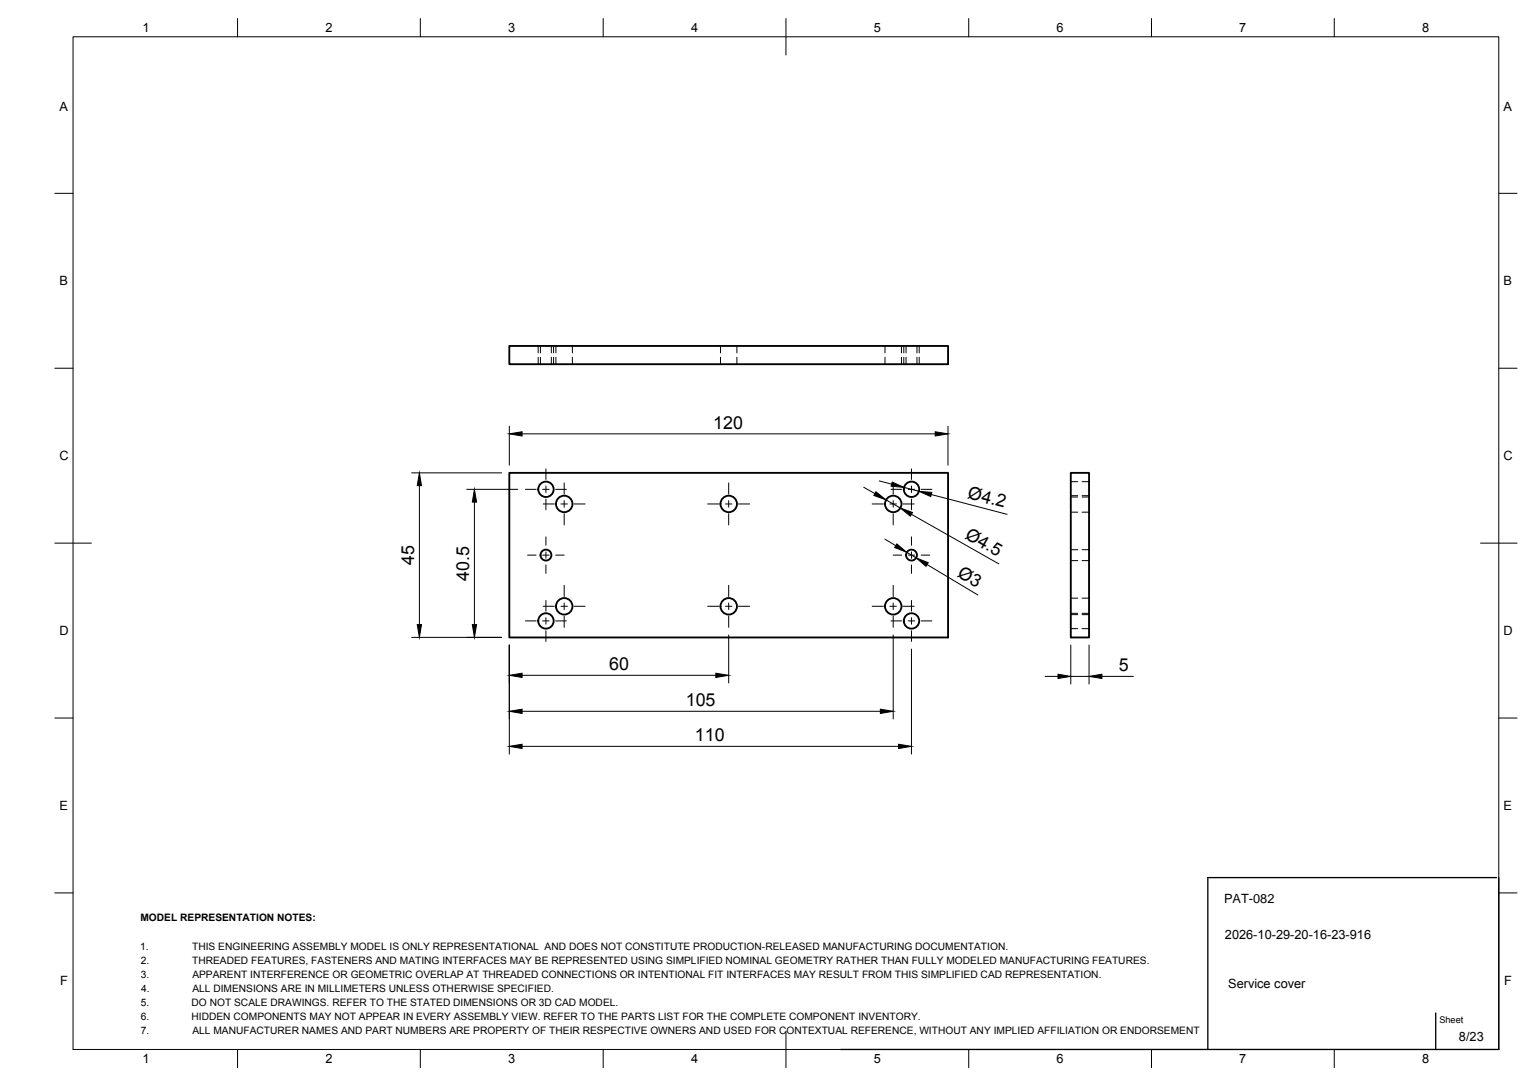
ISO-10303-21;
HEADER;
/* Generated by software containing ST-Developer
 * from STEP Tools, Inc. (www.steptools.com) 
 */

FILE_DESCRIPTION(
/* description */ ('PAT-082'),
/* implementation_level */ '2;1');

FILE_NAME(
/* name */ 'Service cover.step',
/* time_stamp */ '2026-10-29T20:16:13-07:00',
/* author */ (''),
/* organization */ (''),
/* preprocessor_version */ 'ST-DEVELOPER v20.2',
/* originating_system */ 'Autodesk Translation Framework v15.17.0.0',
/* authorisation */ '');

FILE_SCHEMA (('AUTOMOTIVE_DESIGN { 1 0 10303 214 3 1 1 }'));
ENDSEC;

DATA;
#10=MECHANICAL_DESIGN_GEOMETRIC_PRESENTATION_REPRESENTATION('',(#246),#8266);
#202=SHAPE_REPRESENTATION_RELATIONSHIP('SRR','None',#8364,#224);
#224=ADVANCED_BREP_SHAPE_REPRESENTATION('',(#268),#8248);
#246=STYLED_ITEM('',(#8551),#268);
#268=MANIFOLD_SOLID_BREP('Body1',#4586);
#310=FACE_BOUND('',#945,.T.);
#311=FACE_BOUND('',#946,.T.);
#312=FACE_BOUND('',#947,.T.);
#313=FACE_BOUND('',#948,.T.);
#314=FACE_BOUND('',#949,.T.);
#315=FACE_BOUND('',#950,.T.);
#316=FACE_BOUND('',#951,.T.);
#317=FACE_BOUND('',#952,.T.);
#318=FACE_BOUND('',#953,.T.);
#319=FACE_BOUND('',#954,.T.);
#320=FACE_BOUND('',#955,.T.);
#321=FACE_BOUND('',#956,.T.);
#322=FACE_BOUND('',#958,.T.);
#323=FACE_BOUND('',#959,.T.);
#324=FACE_BOUND('',#960,.T.);
#325=FACE_BOUND('',#961,.T.);
#326=FACE_BOUND('',#962,.T.);
#327=FACE_BOUND('',#963,.T.);
#328=FACE_BOUND('',#964,.T.);
#329=FACE_BOUND('',#965,.T.);
#330=FACE_BOUND('',#966,.T.);
#331=FACE_BOUND('',#967,.T.);
#332=FACE_BOUND('',#968,.T.);
#333=FACE_BOUND('',#969,.T.);
#443=PLANE('',#4998);
#444=PLANE('',#4999);
#445=PLANE('',#5000);
#446=PLANE('',#5001);
#447=PLANE('',#5002);
#448=PLANE('',#5003);
#630=FACE_OUTER_BOUND('',#928,.T.);
#631=FACE_OUTER_BOUND('',#929,.T.);
#632=FACE_OUTER_BOUND('',#930,.T.);
#633=FACE_OUTER_BOUND('',#931,.T.);
#634=FACE_OUTER_BOUND('',#932,.T.);
#635=FACE_OUTER_BOUND('',#933,.T.);
#636=FACE_OUTER_BOUND('',#934,.T.);
#637=FACE_OUTER_BOUND('',#935,.T.);
#638=FACE_OUTER_BOUND('',#936,.T.);
#639=FACE_OUTER_BOUND('',#937,.T.);
#640=FACE_OUTER_BOUND('',#938,.T.);
#641=FACE_OUTER_BOUND('',#939,.T.);
#642=FACE_OUTER_BOUND('',#940,.T.);
#643=FACE_OUTER_BOUND('',#941,.T.);
#644=FACE_OUTER_BOUND('',#942,.T.);
#645=FACE_OUTER_BOUND('',#943,.T.);
#646=FACE_OUTER_BOUND('',#944,.T.);
#647=FACE_OUTER_BOUND('',#957,.T.);
#928=EDGE_LOOP('',(#3350,#3351,#3352,#3353));
#929=EDGE_LOOP('',(#3354,#3355,#3356,#3357));
#930=EDGE_LOOP('',(#3358,#3359,#3360,#3361));
#931=EDGE_LOOP('',(#3362,#3363,#3364,#3365));
#932=EDGE_LOOP('',(#3366,#3367,#3368,#3369));
#933=EDGE_LOOP('',(#3370,#3371,#3372,#3373));
#934=EDGE_LOOP('',(#3374,#3375,#3376,#3377));
#935=EDGE_LOOP('',(#3378,#3379,#3380,#3381));
#936=EDGE_LOOP('',(#3382,#3383,#3384,#3385));
#937=EDGE_LOOP('',(#3386,#3387,#3388,#3389));
#938=EDGE_LOOP('',(#3390,#3391,#3392,#3393));
#939=EDGE_LOOP('',(#3394,#3395,#3396,#3397));
#940=EDGE_LOOP('',(#3398,#3399,#3400,#3401));
#941=EDGE_LOOP('',(#3402,#3403,#3404,#3405));
#942=EDGE_LOOP('',(#3406,#3407,#3408,#3409));
#943=EDGE_LOOP('',(#3410,#3411,#3412,#3413));
#944=EDGE_LOOP('',(#3414,#3415,#3416,#3417));
#945=EDGE_LOOP('',(#3418));
#946=EDGE_LOOP('',(#3419));
#947=EDGE_LOOP('',(#3420));
#948=EDGE_LOOP('',(#3421));
#949=EDGE_LOOP('',(#3422));
#950=EDGE_LOOP('',(#3423));
#951=EDGE_LOOP('',(#3424));
#952=EDGE_LOOP('',(#3425));
#953=EDGE_LOOP('',(#3426));
#954=EDGE_LOOP('',(#3427));
#955=EDGE_LOOP('',(#3428));
#956=EDGE_LOOP('',(#3429));
#957=EDGE_LOOP('',(#3430,#3431,#3432,#3433));
#958=EDGE_LOOP('',(#3434));
#959=EDGE_LOOP('',(#3435));
#960=EDGE_LOOP('',(#3436));
#961=EDGE_LOOP('',(#3437));
#962=EDGE_LOOP('',(#3438));
#963=EDGE_LOOP('',(#3439));
#964=EDGE_LOOP('',(#3440));
#965=EDGE_LOOP('',(#3441));
#966=EDGE_LOOP('',(#3442));
#967=EDGE_LOOP('',(#3443));
#968=EDGE_LOOP('',(#3444));
#969=EDGE_LOOP('',(#3445));
#1319=LINE('',#7092,#1674);
#1320=LINE('',#7098,#1675);
#1321=LINE('',#7104,#1676);
#1322=LINE('',#7110,#1677);
#1323=LINE('',#7116,#1678);
#1324=LINE('',#7122,#1679);
#1325=LINE('',#7128,#1680);
#1326=LINE('',#7134,#1681);
#1327=LINE('',#7140,#1682);
#1328=LINE('',#7146,#1683);
#1329=LINE('',#7152,#1684);
#1330=LINE('',#7158,#1685);
#1331=LINE('',#7163,#1686);
#1332=LINE('',#7165,#1687);
#1333=LINE('',#7167,#1688);
#1334=LINE('',#7168,#1689);
#1335=LINE('',#7171,#1690);
#1336=LINE('',#7173,#1691);
#1337=LINE('',#7174,#1692);
#1338=LINE('',#7177,#1693);
#1339=LINE('',#7179,#1694);
#1340=LINE('',#7180,#1695);
#1341=LINE('',#7182,#1696);
#1342=LINE('',#7183,#1697);
#1674=VECTOR('',#5696,0.15);
#1675=VECTOR('',#5703,0.15);
#1676=VECTOR('',#5710,0.225);
#1677=VECTOR('',#5717,0.225);
#1678=VECTOR('',#5724,0.225);
#1679=VECTOR('',#5731,0.225);
#1680=VECTOR('',#5738,0.225);
#1681=VECTOR('',#5745,0.225);
#1682=VECTOR('',#5752,0.21);
#1683=VECTOR('',#5759,0.21);
#1684=VECTOR('',#5766,0.21);
#1685=VECTOR('',#5773,0.21);
#1686=VECTOR('',#5778,1.);
#1687=VECTOR('',#5779,1.);
#1688=VECTOR('',#5780,1.);
#1689=VECTOR('',#5781,1.);
#1690=VECTOR('',#5784,1.);
#1691=VECTOR('',#5785,1.);
#1692=VECTOR('',#5786,1.);
#1693=VECTOR('',#5789,1.);
#1694=VECTOR('',#5790,1.);
#1695=VECTOR('',#5791,1.);
#1696=VECTOR('',#5794,1.);
#1697=VECTOR('',#5795,1.);
#1993=CIRCLE('',#4963,0.15);
#1994=CIRCLE('',#4964,0.15);
#1995=CIRCLE('',#4966,0.15);
#1996=CIRCLE('',#4967,0.15);
#1997=CIRCLE('',#4969,0.225);
#1998=CIRCLE('',#4970,0.225);
#1999=CIRCLE('',#4972,0.225);
#2000=CIRCLE('',#4973,0.225);
#2001=CIRCLE('',#4975,0.225);
#2002=CIRCLE('',#4976,0.225);
#2003=CIRCLE('',#4978,0.225);
#2004=CIRCLE('',#4979,0.225);
#2005=CIRCLE('',#4981,0.225);
#2006=CIRCLE('',#4982,0.225);
#2007=CIRCLE('',#4984,0.225);
#2008=CIRCLE('',#4985,0.225);
#2009=CIRCLE('',#4987,0.21);
#2010=CIRCLE('',#4988,0.21);
#2011=CIRCLE('',#4990,0.21);
#2012=CIRCLE('',#4991,0.21);
#2013=CIRCLE('',#4993,0.21);
#2014=CIRCLE('',#4994,0.21);
#2015=CIRCLE('',#4996,0.21);
#2016=CIRCLE('',#4997,0.21);
#2233=VERTEX_POINT('',#7089);
#2234=VERTEX_POINT('',#7091);
#2235=VERTEX_POINT('',#7095);
#2236=VERTEX_POINT('',#7097);
#2237=VERTEX_POINT('',#7101);
#2238=VERTEX_POINT('',#7103);
#2239=VERTEX_POINT('',#7107);
#2240=VERTEX_POINT('',#7109);
#2241=VERTEX_POINT('',#7113);
#2242=VERTEX_POINT('',#7115);
#2243=VERTEX_POINT('',#7119);
#2244=VERTEX_POINT('',#7121);
#2245=VERTEX_POINT('',#7125);
#2246=VERTEX_POINT('',#7127);
#2247=VERTEX_POINT('',#7131);
#2248=VERTEX_POINT('',#7133);
#2249=VERTEX_POINT('',#7137);
#2250=VERTEX_POINT('',#7139);
#2251=VERTEX_POINT('',#7143);
#2252=VERTEX_POINT('',#7145);
#2253=VERTEX_POINT('',#7149);
#2254=VERTEX_POINT('',#7151);
#2255=VERTEX_POINT('',#7155);
#2256=VERTEX_POINT('',#7157);
#2257=VERTEX_POINT('',#7161);
#2258=VERTEX_POINT('',#7162);
#2259=VERTEX_POINT('',#7164);
#2260=VERTEX_POINT('',#7166);
#2261=VERTEX_POINT('',#7170);
#2262=VERTEX_POINT('',#7172);
#2263=VERTEX_POINT('',#7176);
#2264=VERTEX_POINT('',#7178);
#2651=EDGE_CURVE('',#2233,#2233,#1993,.T.);
#2652=EDGE_CURVE('',#2233,#2234,#1319,.T.);
#2653=EDGE_CURVE('',#2234,#2234,#1994,.T.);
#2654=EDGE_CURVE('',#2235,#2235,#1995,.T.);
#2655=EDGE_CURVE('',#2235,#2236,#1320,.T.);
#2656=EDGE_CURVE('',#2236,#2236,#1996,.T.);
#2657=EDGE_CURVE('',#2237,#2237,#1997,.T.);
#2658=EDGE_CURVE('',#2237,#2238,#1321,.T.);
#2659=EDGE_CURVE('',#2238,#2238,#1998,.T.);
#2660=EDGE_CURVE('',#2239,#2239,#1999,.T.);
#2661=EDGE_CURVE('',#2239,#2240,#1322,.T.);
#2662=EDGE_CURVE('',#2240,#2240,#2000,.T.);
#2663=EDGE_CURVE('',#2241,#2241,#2001,.T.);
#2664=EDGE_CURVE('',#2241,#2242,#1323,.T.);
#2665=EDGE_CURVE('',#2242,#2242,#2002,.T.);
#2666=EDGE_CURVE('',#2243,#2243,#2003,.T.);
#2667=EDGE_CURVE('',#2243,#2244,#1324,.T.);
#2668=EDGE_CURVE('',#2244,#2244,#2004,.T.);
#2669=EDGE_CURVE('',#2245,#2245,#2005,.T.);
#2670=EDGE_CURVE('',#2245,#2246,#1325,.T.);
#2671=EDGE_CURVE('',#2246,#2246,#2006,.T.);
#2672=EDGE_CURVE('',#2247,#2247,#2007,.T.);
#2673=EDGE_CURVE('',#2247,#2248,#1326,.T.);
#2674=EDGE_CURVE('',#2248,#2248,#2008,.T.);
#2675=EDGE_CURVE('',#2249,#2249,#2009,.T.);
#2676=EDGE_CURVE('',#2249,#2250,#1327,.T.);
#2677=EDGE_CURVE('',#2250,#2250,#2010,.T.);
#2678=EDGE_CURVE('',#2251,#2251,#2011,.T.);
#2679=EDGE_CURVE('',#2251,#2252,#1328,.T.);
#2680=EDGE_CURVE('',#2252,#2252,#2012,.T.);
#2681=EDGE_CURVE('',#2253,#2253,#2013,.T.);
#2682=EDGE_CURVE('',#2253,#2254,#1329,.T.);
#2683=EDGE_CURVE('',#2254,#2254,#2014,.T.);
#2684=EDGE_CURVE('',#2255,#2255,#2015,.T.);
#2685=EDGE_CURVE('',#2255,#2256,#1330,.T.);
#2686=EDGE_CURVE('',#2256,#2256,#2016,.T.);
#2687=EDGE_CURVE('',#2257,#2258,#1331,.T.);
#2688=EDGE_CURVE('',#2258,#2259,#1332,.T.);
#2689=EDGE_CURVE('',#2260,#2259,#1333,.T.);
#2690=EDGE_CURVE('',#2257,#2260,#1334,.T.);
#2691=EDGE_CURVE('',#2261,#2257,#1335,.T.);
#2692=EDGE_CURVE('',#2262,#2260,#1336,.T.);
#2693=EDGE_CURVE('',#2261,#2262,#1337,.T.);
#2694=EDGE_CURVE('',#2263,#2261,#1338,.T.);
#2695=EDGE_CURVE('',#2264,#2262,#1339,.T.);
#2696=EDGE_CURVE('',#2263,#2264,#1340,.T.);
#2697=EDGE_CURVE('',#2258,#2263,#1341,.T.);
#2698=EDGE_CURVE('',#2259,#2264,#1342,.T.);
#3350=ORIENTED_EDGE('',*,*,#2651,.F.);
#3351=ORIENTED_EDGE('',*,*,#2652,.T.);
#3352=ORIENTED_EDGE('',*,*,#2653,.F.);
#3353=ORIENTED_EDGE('',*,*,#2652,.F.);
#3354=ORIENTED_EDGE('',*,*,#2654,.F.);
#3355=ORIENTED_EDGE('',*,*,#2655,.T.);
#3356=ORIENTED_EDGE('',*,*,#2656,.F.);
#3357=ORIENTED_EDGE('',*,*,#2655,.F.);
#3358=ORIENTED_EDGE('',*,*,#2657,.F.);
#3359=ORIENTED_EDGE('',*,*,#2658,.T.);
#3360=ORIENTED_EDGE('',*,*,#2659,.F.);
#3361=ORIENTED_EDGE('',*,*,#2658,.F.);
#3362=ORIENTED_EDGE('',*,*,#2660,.F.);
#3363=ORIENTED_EDGE('',*,*,#2661,.T.);
#3364=ORIENTED_EDGE('',*,*,#2662,.F.);
#3365=ORIENTED_EDGE('',*,*,#2661,.F.);
#3366=ORIENTED_EDGE('',*,*,#2663,.F.);
#3367=ORIENTED_EDGE('',*,*,#2664,.T.);
#3368=ORIENTED_EDGE('',*,*,#2665,.F.);
#3369=ORIENTED_EDGE('',*,*,#2664,.F.);
#3370=ORIENTED_EDGE('',*,*,#2666,.F.);
#3371=ORIENTED_EDGE('',*,*,#2667,.T.);
#3372=ORIENTED_EDGE('',*,*,#2668,.F.);
#3373=ORIENTED_EDGE('',*,*,#2667,.F.);
#3374=ORIENTED_EDGE('',*,*,#2669,.F.);
#3375=ORIENTED_EDGE('',*,*,#2670,.T.);
#3376=ORIENTED_EDGE('',*,*,#2671,.F.);
#3377=ORIENTED_EDGE('',*,*,#2670,.F.);
#3378=ORIENTED_EDGE('',*,*,#2672,.F.);
#3379=ORIENTED_EDGE('',*,*,#2673,.T.);
#3380=ORIENTED_EDGE('',*,*,#2674,.F.);
#3381=ORIENTED_EDGE('',*,*,#2673,.F.);
#3382=ORIENTED_EDGE('',*,*,#2675,.F.);
#3383=ORIENTED_EDGE('',*,*,#2676,.T.);
#3384=ORIENTED_EDGE('',*,*,#2677,.F.);
#3385=ORIENTED_EDGE('',*,*,#2676,.F.);
#3386=ORIENTED_EDGE('',*,*,#2678,.F.);
#3387=ORIENTED_EDGE('',*,*,#2679,.T.);
#3388=ORIENTED_EDGE('',*,*,#2680,.F.);
#3389=ORIENTED_EDGE('',*,*,#2679,.F.);
#3390=ORIENTED_EDGE('',*,*,#2681,.F.);
#3391=ORIENTED_EDGE('',*,*,#2682,.T.);
#3392=ORIENTED_EDGE('',*,*,#2683,.F.);
#3393=ORIENTED_EDGE('',*,*,#2682,.F.);
#3394=ORIENTED_EDGE('',*,*,#2684,.F.);
#3395=ORIENTED_EDGE('',*,*,#2685,.T.);
#3396=ORIENTED_EDGE('',*,*,#2686,.F.);
#3397=ORIENTED_EDGE('',*,*,#2685,.F.);
#3398=ORIENTED_EDGE('',*,*,#2687,.T.);
#3399=ORIENTED_EDGE('',*,*,#2688,.T.);
#3400=ORIENTED_EDGE('',*,*,#2689,.F.);
#3401=ORIENTED_EDGE('',*,*,#2690,.F.);
#3402=ORIENTED_EDGE('',*,*,#2691,.T.);
#3403=ORIENTED_EDGE('',*,*,#2690,.T.);
#3404=ORIENTED_EDGE('',*,*,#2692,.F.);
#3405=ORIENTED_EDGE('',*,*,#2693,.F.);
#3406=ORIENTED_EDGE('',*,*,#2694,.T.);
#3407=ORIENTED_EDGE('',*,*,#2693,.T.);
#3408=ORIENTED_EDGE('',*,*,#2695,.F.);
#3409=ORIENTED_EDGE('',*,*,#2696,.F.);
#3410=ORIENTED_EDGE('',*,*,#2697,.T.);
#3411=ORIENTED_EDGE('',*,*,#2696,.T.);
#3412=ORIENTED_EDGE('',*,*,#2698,.F.);
#3413=ORIENTED_EDGE('',*,*,#2688,.F.);
#3414=ORIENTED_EDGE('',*,*,#2698,.T.);
#3415=ORIENTED_EDGE('',*,*,#2695,.T.);
#3416=ORIENTED_EDGE('',*,*,#2692,.T.);
#3417=ORIENTED_EDGE('',*,*,#2689,.T.);
#3418=ORIENTED_EDGE('',*,*,#2656,.T.);
#3419=ORIENTED_EDGE('',*,*,#2686,.T.);
#3420=ORIENTED_EDGE('',*,*,#2683,.T.);
#3421=ORIENTED_EDGE('',*,*,#2680,.T.);
#3422=ORIENTED_EDGE('',*,*,#2677,.T.);
#3423=ORIENTED_EDGE('',*,*,#2674,.T.);
#3424=ORIENTED_EDGE('',*,*,#2671,.T.);
#3425=ORIENTED_EDGE('',*,*,#2668,.T.);
#3426=ORIENTED_EDGE('',*,*,#2665,.T.);
#3427=ORIENTED_EDGE('',*,*,#2662,.T.);
#3428=ORIENTED_EDGE('',*,*,#2659,.T.);
#3429=ORIENTED_EDGE('',*,*,#2653,.T.);
#3430=ORIENTED_EDGE('',*,*,#2697,.F.);
#3431=ORIENTED_EDGE('',*,*,#2687,.F.);
#3432=ORIENTED_EDGE('',*,*,#2691,.F.);
#3433=ORIENTED_EDGE('',*,*,#2694,.F.);
#3434=ORIENTED_EDGE('',*,*,#2654,.T.);
#3435=ORIENTED_EDGE('',*,*,#2684,.T.);
#3436=ORIENTED_EDGE('',*,*,#2681,.T.);
#3437=ORIENTED_EDGE('',*,*,#2678,.T.);
#3438=ORIENTED_EDGE('',*,*,#2675,.T.);
#3439=ORIENTED_EDGE('',*,*,#2672,.T.);
#3440=ORIENTED_EDGE('',*,*,#2669,.T.);
#3441=ORIENTED_EDGE('',*,*,#2666,.T.);
#3442=ORIENTED_EDGE('',*,*,#2663,.T.);
#3443=ORIENTED_EDGE('',*,*,#2660,.T.);
#3444=ORIENTED_EDGE('',*,*,#2657,.T.);
#3445=ORIENTED_EDGE('',*,*,#2651,.T.);
#4240=CYLINDRICAL_SURFACE('',#4962,0.15);
#4241=CYLINDRICAL_SURFACE('',#4965,0.15);
#4242=CYLINDRICAL_SURFACE('',#4968,0.225);
#4243=CYLINDRICAL_SURFACE('',#4971,0.225);
#4244=CYLINDRICAL_SURFACE('',#4974,0.225);
#4245=CYLINDRICAL_SURFACE('',#4977,0.225);
#4246=CYLINDRICAL_SURFACE('',#4980,0.225);
#4247=CYLINDRICAL_SURFACE('',#4983,0.225);
#4248=CYLINDRICAL_SURFACE('',#4986,0.21);
#4249=CYLINDRICAL_SURFACE('',#4989,0.21);
#4250=CYLINDRICAL_SURFACE('',#4992,0.21);
#4251=CYLINDRICAL_SURFACE('',#4995,0.21);
#4369=ADVANCED_FACE('',(#630),#4240,.F.);
#4370=ADVANCED_FACE('',(#631),#4241,.F.);
#4371=ADVANCED_FACE('',(#632),#4242,.F.);
#4372=ADVANCED_FACE('',(#633),#4243,.F.);
#4373=ADVANCED_FACE('',(#634),#4244,.F.);
#4374=ADVANCED_FACE('',(#635),#4245,.F.);
#4375=ADVANCED_FACE('',(#636),#4246,.F.);
#4376=ADVANCED_FACE('',(#637),#4247,.F.);
#4377=ADVANCED_FACE('',(#638),#4248,.F.);
#4378=ADVANCED_FACE('',(#639),#4249,.F.);
#4379=ADVANCED_FACE('',(#640),#4250,.F.);
#4380=ADVANCED_FACE('',(#641),#4251,.F.);
#4381=ADVANCED_FACE('',(#642),#443,.T.);
#4382=ADVANCED_FACE('',(#643),#444,.T.);
#4383=ADVANCED_FACE('',(#644),#445,.T.);
#4384=ADVANCED_FACE('',(#645),#446,.T.);
#4385=ADVANCED_FACE('',(#646,#310,#311,#312,#313,#314,#315,#316,#317,#318,
#319,#320,#321),#447,.T.);
#4386=ADVANCED_FACE('',(#647,#322,#323,#324,#325,#326,#327,#328,#329,#330,
#331,#332,#333),#448,.F.);
#4586=CLOSED_SHELL('',(#4369,#4370,#4371,#4372,#4373,#4374,#4375,#4376,
#4377,#4378,#4379,#4380,#4381,#4382,#4383,#4384,#4385,#4386));
#4961=AXIS2_PLACEMENT_3D('',#7087,#5690,#5691);
#4962=AXIS2_PLACEMENT_3D('',#7088,#5692,#5693);
#4963=AXIS2_PLACEMENT_3D('',#7090,#5694,#5695);
#4964=AXIS2_PLACEMENT_3D('',#7093,#5697,#5698);
#4965=AXIS2_PLACEMENT_3D('',#7094,#5699,#5700);
#4966=AXIS2_PLACEMENT_3D('',#7096,#5701,#5702);
#4967=AXIS2_PLACEMENT_3D('',#7099,#5704,#5705);
#4968=AXIS2_PLACEMENT_3D('',#7100,#5706,#5707);
#4969=AXIS2_PLACEMENT_3D('',#7102,#5708,#5709);
#4970=AXIS2_PLACEMENT_3D('',#7105,#5711,#5712);
#4971=AXIS2_PLACEMENT_3D('',#7106,#5713,#5714);
#4972=AXIS2_PLACEMENT_3D('',#7108,#5715,#5716);
#4973=AXIS2_PLACEMENT_3D('',#7111,#5718,#5719);
#4974=AXIS2_PLACEMENT_3D('',#7112,#5720,#5721);
#4975=AXIS2_PLACEMENT_3D('',#7114,#5722,#5723);
#4976=AXIS2_PLACEMENT_3D('',#7117,#5725,#5726);
#4977=AXIS2_PLACEMENT_3D('',#7118,#5727,#5728);
#4978=AXIS2_PLACEMENT_3D('',#7120,#5729,#5730);
#4979=AXIS2_PLACEMENT_3D('',#7123,#5732,#5733);
#4980=AXIS2_PLACEMENT_3D('',#7124,#5734,#5735);
#4981=AXIS2_PLACEMENT_3D('',#7126,#5736,#5737);
#4982=AXIS2_PLACEMENT_3D('',#7129,#5739,#5740);
#4983=AXIS2_PLACEMENT_3D('',#7130,#5741,#5742);
#4984=AXIS2_PLACEMENT_3D('',#7132,#5743,#5744);
#4985=AXIS2_PLACEMENT_3D('',#7135,#5746,#5747);
#4986=AXIS2_PLACEMENT_3D('',#7136,#5748,#5749);
#4987=AXIS2_PLACEMENT_3D('',#7138,#5750,#5751);
#4988=AXIS2_PLACEMENT_3D('',#7141,#5753,#5754);
#4989=AXIS2_PLACEMENT_3D('',#7142,#5755,#5756);
#4990=AXIS2_PLACEMENT_3D('',#7144,#5757,#5758);
#4991=AXIS2_PLACEMENT_3D('',#7147,#5760,#5761);
#4992=AXIS2_PLACEMENT_3D('',#7148,#5762,#5763);
#4993=AXIS2_PLACEMENT_3D('',#7150,#5764,#5765);
#4994=AXIS2_PLACEMENT_3D('',#7153,#5767,#5768);
#4995=AXIS2_PLACEMENT_3D('',#7154,#5769,#5770);
#4996=AXIS2_PLACEMENT_3D('',#7156,#5771,#5772);
#4997=AXIS2_PLACEMENT_3D('',#7159,#5774,#5775);
#4998=AXIS2_PLACEMENT_3D('',#7160,#5776,#5777);
#4999=AXIS2_PLACEMENT_3D('',#7169,#5782,#5783);
#5000=AXIS2_PLACEMENT_3D('',#7175,#5787,#5788);
#5001=AXIS2_PLACEMENT_3D('',#7181,#5792,#5793);
#5002=AXIS2_PLACEMENT_3D('',#7184,#5796,#5797);
#5003=AXIS2_PLACEMENT_3D('',#7185,#5798,#5799);
#5690=DIRECTION('axis',(0.,0.,1.));
#5691=DIRECTION('refdir',(1.,0.,0.));
#5692=DIRECTION('center_axis',(0.,0.,1.));
#5693=DIRECTION('ref_axis',(1.,0.,0.));
#5694=DIRECTION('center_axis',(0.,0.,1.));
#5695=DIRECTION('ref_axis',(1.,0.,0.));
#5696=DIRECTION('',(0.,0.,1.));
#5697=DIRECTION('center_axis',(0.,0.,-1.));
#5698=DIRECTION('ref_axis',(1.,0.,0.));
#5699=DIRECTION('center_axis',(0.,0.,1.));
#5700=DIRECTION('ref_axis',(1.,0.,0.));
#5701=DIRECTION('center_axis',(0.,0.,1.));
#5702=DIRECTION('ref_axis',(1.,0.,0.));
#5703=DIRECTION('',(0.,0.,1.));
#5704=DIRECTION('center_axis',(0.,0.,-1.));
#5705=DIRECTION('ref_axis',(1.,0.,0.));
#5706=DIRECTION('center_axis',(0.,0.,1.));
#5707=DIRECTION('ref_axis',(1.,0.,0.));
#5708=DIRECTION('center_axis',(0.,0.,1.));
#5709=DIRECTION('ref_axis',(1.,0.,0.));
#5710=DIRECTION('',(0.,0.,1.));
#5711=DIRECTION('center_axis',(0.,0.,-1.));
#5712=DIRECTION('ref_axis',(1.,0.,0.));
#5713=DIRECTION('center_axis',(0.,0.,1.));
#5714=DIRECTION('ref_axis',(1.,0.,0.));
#5715=DIRECTION('center_axis',(0.,0.,1.));
#5716=DIRECTION('ref_axis',(1.,0.,0.));
#5717=DIRECTION('',(0.,0.,1.));
#5718=DIRECTION('center_axis',(0.,0.,-1.));
#5719=DIRECTION('ref_axis',(1.,0.,0.));
#5720=DIRECTION('center_axis',(0.,0.,1.));
#5721=DIRECTION('ref_axis',(1.,0.,0.));
#5722=DIRECTION('center_axis',(0.,0.,1.));
#5723=DIRECTION('ref_axis',(1.,0.,0.));
#5724=DIRECTION('',(0.,0.,1.));
#5725=DIRECTION('center_axis',(0.,0.,-1.));
#5726=DIRECTION('ref_axis',(1.,0.,0.));
#5727=DIRECTION('center_axis',(0.,0.,1.));
#5728=DIRECTION('ref_axis',(1.,0.,0.));
#5729=DIRECTION('center_axis',(0.,0.,1.));
#5730=DIRECTION('ref_axis',(1.,0.,0.));
#5731=DIRECTION('',(0.,0.,1.));
#5732=DIRECTION('center_axis',(0.,0.,-1.));
#5733=DIRECTION('ref_axis',(1.,0.,0.));
#5734=DIRECTION('center_axis',(0.,0.,1.));
#5735=DIRECTION('ref_axis',(1.,0.,0.));
#5736=DIRECTION('center_axis',(0.,0.,1.));
#5737=DIRECTION('ref_axis',(1.,0.,0.));
#5738=DIRECTION('',(0.,0.,1.));
#5739=DIRECTION('center_axis',(0.,0.,-1.));
#5740=DIRECTION('ref_axis',(1.,0.,0.));
#5741=DIRECTION('center_axis',(0.,0.,1.));
#5742=DIRECTION('ref_axis',(1.,0.,0.));
#5743=DIRECTION('center_axis',(0.,0.,1.));
#5744=DIRECTION('ref_axis',(1.,0.,0.));
#5745=DIRECTION('',(0.,0.,1.));
#5746=DIRECTION('center_axis',(0.,0.,-1.));
#5747=DIRECTION('ref_axis',(1.,0.,0.));
#5748=DIRECTION('center_axis',(0.,0.,1.));
#5749=DIRECTION('ref_axis',(1.,0.,0.));
#5750=DIRECTION('center_axis',(0.,0.,1.));
#5751=DIRECTION('ref_axis',(1.,0.,0.));
#5752=DIRECTION('',(0.,0.,1.));
#5753=DIRECTION('center_axis',(0.,0.,-1.));
#5754=DIRECTION('ref_axis',(1.,0.,0.));
#5755=DIRECTION('center_axis',(0.,0.,1.));
#5756=DIRECTION('ref_axis',(1.,0.,0.));
#5757=DIRECTION('center_axis',(0.,0.,1.));
#5758=DIRECTION('ref_axis',(1.,0.,0.));
#5759=DIRECTION('',(0.,0.,1.));
#5760=DIRECTION('center_axis',(0.,0.,-1.));
#5761=DIRECTION('ref_axis',(1.,0.,0.));
#5762=DIRECTION('center_axis',(0.,0.,1.));
#5763=DIRECTION('ref_axis',(1.,0.,0.));
#5764=DIRECTION('center_axis',(0.,0.,1.));
#5765=DIRECTION('ref_axis',(1.,0.,0.));
#5766=DIRECTION('',(0.,0.,1.));
#5767=DIRECTION('center_axis',(0.,0.,-1.));
#5768=DIRECTION('ref_axis',(1.,0.,0.));
#5769=DIRECTION('center_axis',(0.,0.,1.));
#5770=DIRECTION('ref_axis',(1.,0.,0.));
#5771=DIRECTION('center_axis',(0.,0.,1.));
#5772=DIRECTION('ref_axis',(1.,0.,0.));
#5773=DIRECTION('',(0.,0.,1.));
#5774=DIRECTION('center_axis',(0.,0.,-1.));
#5775=DIRECTION('ref_axis',(1.,0.,0.));
#5776=DIRECTION('center_axis',(0.,1.,0.));
#5777=DIRECTION('ref_axis',(-1.,0.,0.));
#5778=DIRECTION('',(-1.,0.,0.));
#5779=DIRECTION('',(0.,0.,1.));
#5780=DIRECTION('',(-1.,0.,0.));
#5781=DIRECTION('',(0.,0.,1.));
#5782=DIRECTION('center_axis',(1.,0.,0.));
#5783=DIRECTION('ref_axis',(0.,1.,0.));
#5784=DIRECTION('',(0.,1.,0.));
#5785=DIRECTION('',(0.,1.,0.));
#5786=DIRECTION('',(0.,0.,1.));
#5787=DIRECTION('center_axis',(0.,-1.,0.));
#5788=DIRECTION('ref_axis',(1.,0.,0.));
#5789=DIRECTION('',(1.,0.,0.));
#5790=DIRECTION('',(1.,0.,0.));
#5791=DIRECTION('',(0.,0.,1.));
#5792=DIRECTION('center_axis',(-1.,0.,0.));
#5793=DIRECTION('ref_axis',(0.,-1.,0.));
#5794=DIRECTION('',(0.,-1.,0.));
#5795=DIRECTION('',(0.,-1.,0.));
#5796=DIRECTION('center_axis',(0.,0.,1.));
#5797=DIRECTION('ref_axis',(1.,0.,0.));
#5798=DIRECTION('center_axis',(0.,0.,1.));
#5799=DIRECTION('ref_axis',(1.,0.,0.));
#7087=CARTESIAN_POINT('',(0.,0.,0.));
#7088=CARTESIAN_POINT('Origin',(5.,0.,1.3));
#7089=CARTESIAN_POINT('',(4.85,-1.83697019872103E-17,1.4));
#7090=CARTESIAN_POINT('Origin',(5.,0.,1.4));
#7091=CARTESIAN_POINT('',(4.85,1.83697019872103E-17,1.9));
#7092=CARTESIAN_POINT('',(4.85,-1.83697019872103E-17,1.3));
#7093=CARTESIAN_POINT('Origin',(5.,0.,1.9));
#7094=CARTESIAN_POINT('Origin',(-5.,0.,1.3));
#7095=CARTESIAN_POINT('',(-5.15,-1.83697019872103E-17,1.4));
#7096=CARTESIAN_POINT('Origin',(-5.,0.,1.4));
#7097=CARTESIAN_POINT('',(-5.15,1.83697019872103E-17,1.9));
#7098=CARTESIAN_POINT('',(-5.15,-1.83697019872103E-17,1.3));
#7099=CARTESIAN_POINT('Origin',(-5.,0.,1.9));
#7100=CARTESIAN_POINT('Origin',(4.5,-1.4,1.3));
#7101=CARTESIAN_POINT('',(4.275,-1.4,1.4));
#7102=CARTESIAN_POINT('Origin',(4.5,-1.4,1.4));
#7103=CARTESIAN_POINT('',(4.275,-1.4,1.9));
#7104=CARTESIAN_POINT('',(4.275,-1.4,1.3));
#7105=CARTESIAN_POINT('Origin',(4.5,-1.4,1.9));
#7106=CARTESIAN_POINT('Origin',(-4.5,-1.4,1.3));
#7107=CARTESIAN_POINT('',(-4.725,-1.4,1.4));
#7108=CARTESIAN_POINT('Origin',(-4.5,-1.4,1.4));
#7109=CARTESIAN_POINT('',(-4.725,-1.4,1.9));
#7110=CARTESIAN_POINT('',(-4.725,-1.4,1.3));
#7111=CARTESIAN_POINT('Origin',(-4.5,-1.4,1.9));
#7112=CARTESIAN_POINT('Origin',(-4.5,1.4,1.3));
#7113=CARTESIAN_POINT('',(-4.725,1.4,1.4));
#7114=CARTESIAN_POINT('Origin',(-4.5,1.4,1.4));
#7115=CARTESIAN_POINT('',(-4.725,1.4,1.9));
#7116=CARTESIAN_POINT('',(-4.725,1.4,1.3));
#7117=CARTESIAN_POINT('Origin',(-4.5,1.4,1.9));
#7118=CARTESIAN_POINT('Origin',(0.,-1.4,1.3));
#7119=CARTESIAN_POINT('',(-0.225,-1.4,1.4));
#7120=CARTESIAN_POINT('Origin',(0.,-1.4,1.4));
#7121=CARTESIAN_POINT('',(-0.225,-1.4,1.9));
#7122=CARTESIAN_POINT('',(-0.225,-1.4,1.3));
#7123=CARTESIAN_POINT('Origin',(0.,-1.4,1.9));
#7124=CARTESIAN_POINT('Origin',(0.,1.4,1.3));
#7125=CARTESIAN_POINT('',(-0.225,1.4,1.4));
#7126=CARTESIAN_POINT('Origin',(0.,1.4,1.4));
#7127=CARTESIAN_POINT('',(-0.225,1.4,1.9));
#7128=CARTESIAN_POINT('',(-0.225,1.4,1.3));
#7129=CARTESIAN_POINT('Origin',(0.,1.4,1.9));
#7130=CARTESIAN_POINT('Origin',(4.5,1.4,1.3));
#7131=CARTESIAN_POINT('',(4.275,1.4,1.4));
#7132=CARTESIAN_POINT('Origin',(4.5,1.4,1.4));
#7133=CARTESIAN_POINT('',(4.275,1.4,1.9));
#7134=CARTESIAN_POINT('',(4.275,1.4,1.3));
#7135=CARTESIAN_POINT('Origin',(4.5,1.4,1.9));
#7136=CARTESIAN_POINT('Origin',(5.,-1.8,1.3));
#7137=CARTESIAN_POINT('',(4.79,-1.8,1.4));
#7138=CARTESIAN_POINT('Origin',(5.,-1.8,1.4));
#7139=CARTESIAN_POINT('',(4.79,-1.8,1.9));
#7140=CARTESIAN_POINT('',(4.79,-1.8,1.3));
#7141=CARTESIAN_POINT('Origin',(5.,-1.8,1.9));
#7142=CARTESIAN_POINT('Origin',(-5.,1.8,1.3));
#7143=CARTESIAN_POINT('',(-5.21,1.8,1.4));
#7144=CARTESIAN_POINT('Origin',(-5.,1.8,1.4));
#7145=CARTESIAN_POINT('',(-5.21,1.8,1.9));
#7146=CARTESIAN_POINT('',(-5.21,1.8,1.3));
#7147=CARTESIAN_POINT('Origin',(-5.,1.8,1.9));
#7148=CARTESIAN_POINT('Origin',(-5.,-1.8,1.3));
#7149=CARTESIAN_POINT('',(-5.21,-1.8,1.4));
#7150=CARTESIAN_POINT('Origin',(-5.,-1.8,1.4));
#7151=CARTESIAN_POINT('',(-5.21,-1.8,1.9));
#7152=CARTESIAN_POINT('',(-5.21,-1.8,1.3));
#7153=CARTESIAN_POINT('Origin',(-5.,-1.8,1.9));
#7154=CARTESIAN_POINT('Origin',(5.,1.8,1.3));
#7155=CARTESIAN_POINT('',(4.79,1.8,1.4));
#7156=CARTESIAN_POINT('Origin',(5.,1.8,1.4));
#7157=CARTESIAN_POINT('',(4.79,1.8,1.9));
#7158=CARTESIAN_POINT('',(4.79,1.8,1.3));
#7159=CARTESIAN_POINT('Origin',(5.,1.8,1.9));
#7160=CARTESIAN_POINT('Origin',(6.,2.25,1.4));
#7161=CARTESIAN_POINT('',(6.,2.25,1.4));
#7162=CARTESIAN_POINT('',(-6.,2.25,1.4));
#7163=CARTESIAN_POINT('',(6.,2.25,1.4));
#7164=CARTESIAN_POINT('',(-6.,2.25,1.9));
#7165=CARTESIAN_POINT('',(-6.,2.25,1.4));
#7166=CARTESIAN_POINT('',(6.,2.25,1.9));
#7167=CARTESIAN_POINT('',(6.,2.25,1.9));
#7168=CARTESIAN_POINT('',(6.,2.25,1.4));
#7169=CARTESIAN_POINT('Origin',(6.,-2.25,1.4));
#7170=CARTESIAN_POINT('',(6.,-2.25,1.4));
#7171=CARTESIAN_POINT('',(6.,-2.25,1.4));
#7172=CARTESIAN_POINT('',(6.,-2.25,1.9));
#7173=CARTESIAN_POINT('',(6.,-2.25,1.9));
#7174=CARTESIAN_POINT('',(6.,-2.25,1.4));
#7175=CARTESIAN_POINT('Origin',(-6.,-2.25,1.4));
#7176=CARTESIAN_POINT('',(-6.,-2.25,1.4));
#7177=CARTESIAN_POINT('',(-6.,-2.25,1.4));
#7178=CARTESIAN_POINT('',(-6.,-2.25,1.9));
#7179=CARTESIAN_POINT('',(-6.,-2.25,1.9));
#7180=CARTESIAN_POINT('',(-6.,-2.25,1.4));
#7181=CARTESIAN_POINT('Origin',(-6.,2.25,1.4));
#7182=CARTESIAN_POINT('',(-6.,2.25,1.4));
#7183=CARTESIAN_POINT('',(-6.,2.25,1.9));
#7184=CARTESIAN_POINT('Origin',(0.,0.,1.9));
#7185=CARTESIAN_POINT('Origin',(0.,0.,1.4));
#8223=UNCERTAINTY_MEASURE_WITH_UNIT(LENGTH_MEASURE(0.001),#8267,
'DISTANCE_ACCURACY_VALUE',
'Maximum model space distance between geometric entities at asserted c
onnectivities');
#8241=UNCERTAINTY_MEASURE_WITH_UNIT(LENGTH_MEASURE(0.001),#8267,
'DISTANCE_ACCURACY_VALUE',
'Maximum model space distance between geometric entities at asserted c
onnectivities');
#8248=(
GEOMETRIC_REPRESENTATION_CONTEXT(3)
GLOBAL_UNCERTAINTY_ASSIGNED_CONTEXT((#8223))
GLOBAL_UNIT_ASSIGNED_CONTEXT((#8267,#8269,#8270))
REPRESENTATION_CONTEXT('','3D')
);
#8266=(
GEOMETRIC_REPRESENTATION_CONTEXT(3)
GLOBAL_UNCERTAINTY_ASSIGNED_CONTEXT((#8241))
GLOBAL_UNIT_ASSIGNED_CONTEXT((#8267,#8269,#8270))
REPRESENTATION_CONTEXT('','3D')
);
#8267=(
LENGTH_UNIT()
NAMED_UNIT(*)
SI_UNIT(.CENTI.,.METRE.)
);
#8269=(
NAMED_UNIT(*)
PLANE_ANGLE_UNIT()
SI_UNIT($,.RADIAN.)
);
#8270=(
NAMED_UNIT(*)
SI_UNIT($,.STERADIAN.)
SOLID_ANGLE_UNIT()
);
#8277=SHAPE_DEFINITION_REPRESENTATION(#8301,#8364);
#8301=PRODUCT_DEFINITION_SHAPE('',$,#8389);
#8364=SHAPE_REPRESENTATION('',(#4961),#8248);
#8382=PRODUCT_DEFINITION_CONTEXT('part definition',#8456,'design');
#8389=PRODUCT_DEFINITION('Service cover','Service cover',#8413,
#8382);
#8413=PRODUCT_DEFINITION_FORMATION('',$,#8464);
#8456=APPLICATION_CONTEXT(
'Core Data for Automotive Mechanical Design Process');
#8457=PRODUCT_CONTEXT('part definition',#8456,'mechanical');
#8464=PRODUCT('Service cover','Service cover',
'Service cover',(#8457));
#8545=COLOUR_RGB('Off White',0.89,0.88,0.83);
#8546=FILL_AREA_STYLE_COLOUR('',#8545);
#8547=FILL_AREA_STYLE('',(#8546));
#8548=SURFACE_STYLE_FILL_AREA(#8547);
#8549=SURFACE_SIDE_STYLE('',(#8548));
#8550=SURFACE_STYLE_USAGE(.BOTH.,#8549);
#8551=PRESENTATION_STYLE_ASSIGNMENT((#8550));
ENDSEC;
END-ISO-10303-21;
